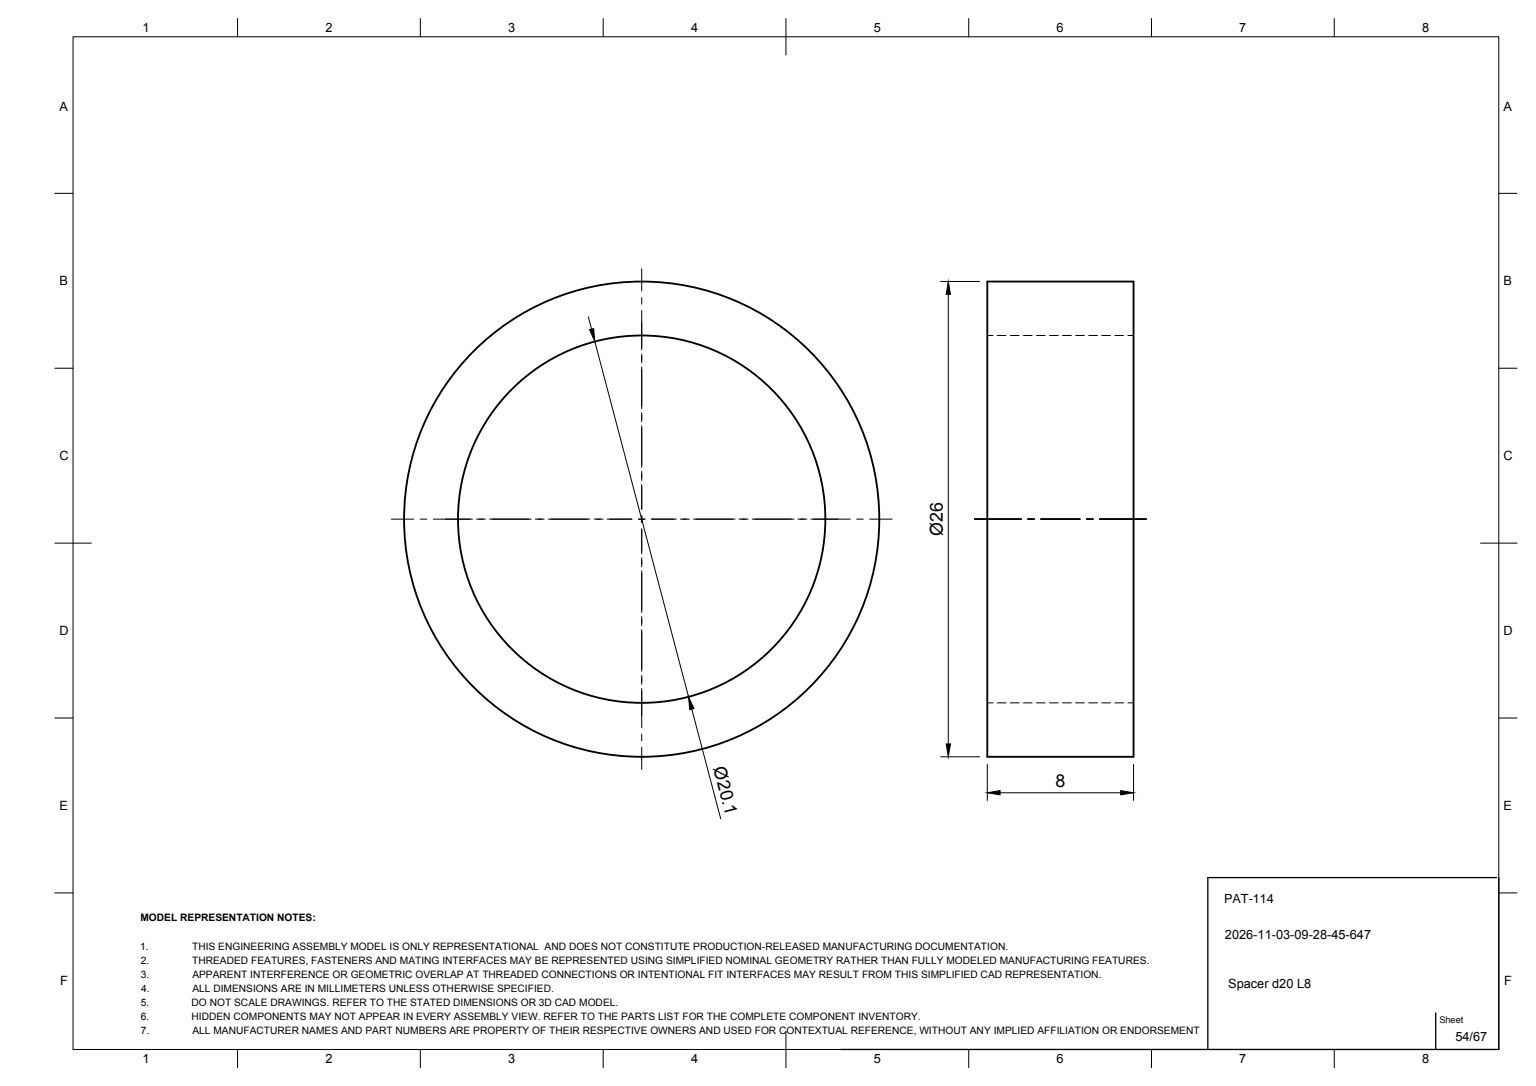
ISO-10303-21;
HEADER;
/* Generated by software containing ST-Developer
 * from STEP Tools, Inc. (www.steptools.com) 
 */

FILE_DESCRIPTION(
/* description */ ('Two-stage gear reducer in split housing'),
/* implementation_level */ '2;1');

FILE_NAME(
/* name */ 'Spacer d20 L8.step',
/* time_stamp */ '2026-10-28T03:22:31-07:00',
/* author */ (''),
/* organization */ (''),
/* preprocessor_version */ 'ST-DEVELOPER v20.2',
/* originating_system */ 'Autodesk Translation Framework v15.17.0.0',
/* authorisation */ '');

FILE_SCHEMA (('AUTOMOTIVE_DESIGN { 1 0 10303 214 3 1 1 }'));
ENDSEC;

DATA;
#10=MECHANICAL_DESIGN_GEOMETRIC_PRESENTATION_REPRESENTATION('',(#1292),#73366);
#1165=SHAPE_REPRESENTATION_RELATIONSHIP('SRR','None',#73656,#1221);
#1221=ADVANCED_BREP_SHAPE_REPRESENTATION('',(#1361),#73352);
#1292=STYLED_ITEM('',(#73981),#1361);
#1361=MANIFOLD_SOLID_BREP('Body1',#16182);
#1574=FACE_BOUND('',#3707,.T.);
#1575=FACE_BOUND('',#3709,.T.);
#1884=PLANE('',#18033);
#1885=PLANE('',#18034);
#2591=FACE_OUTER_BOUND('',#3704,.T.);
#2592=FACE_OUTER_BOUND('',#3705,.T.);
#2593=FACE_OUTER_BOUND('',#3706,.T.);
#2594=FACE_OUTER_BOUND('',#3708,.T.);
#3704=EDGE_LOOP('',(#13143,#13144,#13145,#13146));
#3705=EDGE_LOOP('',(#13147,#13148,#13149,#13150));
#3706=EDGE_LOOP('',(#13151));
#3707=EDGE_LOOP('',(#13152));
#3708=EDGE_LOOP('',(#13153));
#3709=EDGE_LOOP('',(#13154));
#4700=LINE('',#37636,#5724);
#4701=LINE('',#37642,#5725);
#5724=VECTOR('',#21536,1.005);
#5725=VECTOR('',#21543,1.3);
#6650=CIRCLE('',#18028,1.005);
#6651=CIRCLE('',#18029,1.005);
#6652=CIRCLE('',#18031,1.3);
#6653=CIRCLE('',#18032,1.3);
#7719=VERTEX_POINT('',#37633);
#7720=VERTEX_POINT('',#37635);
#7721=VERTEX_POINT('',#37639);
#7722=VERTEX_POINT('',#37641);
#9625=EDGE_CURVE('',#7719,#7719,#6650,.T.);
#9626=EDGE_CURVE('',#7719,#7720,#4700,.T.);
#9627=EDGE_CURVE('',#7720,#7720,#6651,.T.);
#9628=EDGE_CURVE('',#7721,#7721,#6652,.T.);
#9629=EDGE_CURVE('',#7721,#7722,#4701,.T.);
#9630=EDGE_CURVE('',#7722,#7722,#6653,.T.);
#13143=ORIENTED_EDGE('',*,*,#9625,.F.);
#13144=ORIENTED_EDGE('',*,*,#9626,.T.);
#13145=ORIENTED_EDGE('',*,*,#9627,.T.);
#13146=ORIENTED_EDGE('',*,*,#9626,.F.);
#13147=ORIENTED_EDGE('',*,*,#9628,.F.);
#13148=ORIENTED_EDGE('',*,*,#9629,.T.);
#13149=ORIENTED_EDGE('',*,*,#9630,.T.);
#13150=ORIENTED_EDGE('',*,*,#9629,.F.);
#13151=ORIENTED_EDGE('',*,*,#9628,.T.);
#13152=ORIENTED_EDGE('',*,*,#9625,.T.);
#13153=ORIENTED_EDGE('',*,*,#9630,.F.);
#13154=ORIENTED_EDGE('',*,*,#9627,.F.);
#15125=CYLINDRICAL_SURFACE('',#18027,1.005);
#15126=CYLINDRICAL_SURFACE('',#18030,1.3);
#15798=ADVANCED_FACE('',(#2591),#15125,.F.);
#15799=ADVANCED_FACE('',(#2592),#15126,.T.);
#15800=ADVANCED_FACE('',(#2593,#1574),#1884,.T.);
#15801=ADVANCED_FACE('',(#2594,#1575),#1885,.F.);
#16182=CLOSED_SHELL('',(#15798,#15799,#15800,#15801));
#18026=AXIS2_PLACEMENT_3D('',#37631,#21530,#21531);
#18027=AXIS2_PLACEMENT_3D('',#37632,#21532,#21533);
#18028=AXIS2_PLACEMENT_3D('',#37634,#21534,#21535);
#18029=AXIS2_PLACEMENT_3D('',#37637,#21537,#21538);
#18030=AXIS2_PLACEMENT_3D('',#37638,#21539,#21540);
#18031=AXIS2_PLACEMENT_3D('',#37640,#21541,#21542);
#18032=AXIS2_PLACEMENT_3D('',#37643,#21544,#21545);
#18033=AXIS2_PLACEMENT_3D('',#37644,#21546,#21547);
#18034=AXIS2_PLACEMENT_3D('',#37645,#21548,#21549);
#21530=DIRECTION('axis',(0.,0.,1.));
#21531=DIRECTION('refdir',(1.,0.,0.));
#21532=DIRECTION('center_axis',(0.,1.,0.));
#21533=DIRECTION('ref_axis',(1.,0.,0.));
#21534=DIRECTION('center_axis',(0.,-1.,0.));
#21535=DIRECTION('ref_axis',(1.,0.,0.));
#21536=DIRECTION('',(0.,-1.,0.));
#21537=DIRECTION('center_axis',(0.,-1.,0.));
#21538=DIRECTION('ref_axis',(1.,0.,0.));
#21539=DIRECTION('center_axis',(0.,1.,0.));
#21540=DIRECTION('ref_axis',(1.,0.,0.));
#21541=DIRECTION('center_axis',(0.,1.,0.));
#21542=DIRECTION('ref_axis',(1.,0.,0.));
#21543=DIRECTION('',(0.,-1.,0.));
#21544=DIRECTION('center_axis',(0.,1.,0.));
#21545=DIRECTION('ref_axis',(1.,0.,0.));
#21546=DIRECTION('center_axis',(0.,1.,0.));
#21547=DIRECTION('ref_axis',(1.,0.,0.));
#21548=DIRECTION('center_axis',(0.,1.,0.));
#21549=DIRECTION('ref_axis',(1.,0.,0.));
#37631=CARTESIAN_POINT('',(0.,0.,0.));
#37632=CARTESIAN_POINT('Origin',(6.,0.2,10.));
#37633=CARTESIAN_POINT('',(4.995,1.,10.));
#37634=CARTESIAN_POINT('Origin',(6.,1.,10.));
#37635=CARTESIAN_POINT('',(4.995,0.2,10.));
#37636=CARTESIAN_POINT('',(4.995,0.2,10.));
#37637=CARTESIAN_POINT('Origin',(6.,0.2,10.));
#37638=CARTESIAN_POINT('Origin',(6.,0.2,10.));
#37639=CARTESIAN_POINT('',(4.7,1.,10.));
#37640=CARTESIAN_POINT('Origin',(6.,1.,10.));
#37641=CARTESIAN_POINT('',(4.7,0.2,10.));
#37642=CARTESIAN_POINT('',(4.7,0.2,10.));
#37643=CARTESIAN_POINT('Origin',(6.,0.2,10.));
#37644=CARTESIAN_POINT('Origin',(6.,1.,10.));
#37645=CARTESIAN_POINT('Origin',(6.,0.2,10.));
#73288=UNCERTAINTY_MEASURE_WITH_UNIT(LENGTH_MEASURE(0.001),#73367,
'DISTANCE_ACCURACY_VALUE',
'Maximum model space distance between geometric entities at asserted c
onnectivities');
#73302=UNCERTAINTY_MEASURE_WITH_UNIT(LENGTH_MEASURE(0.001),#73367,
'DISTANCE_ACCURACY_VALUE',
'Maximum model space distance between geometric entities at asserted c
onnectivities');
#73352=(
GEOMETRIC_REPRESENTATION_CONTEXT(3)
GLOBAL_UNCERTAINTY_ASSIGNED_CONTEXT((#73288))
GLOBAL_UNIT_ASSIGNED_CONTEXT((#73367,#73369,#73370))
REPRESENTATION_CONTEXT('','3D')
);
#73366=(
GEOMETRIC_REPRESENTATION_CONTEXT(3)
GLOBAL_UNCERTAINTY_ASSIGNED_CONTEXT((#73302))
GLOBAL_UNIT_ASSIGNED_CONTEXT((#73367,#73369,#73370))
REPRESENTATION_CONTEXT('','3D')
);
#73367=(
LENGTH_UNIT()
NAMED_UNIT(*)
SI_UNIT(.CENTI.,.METRE.)
);
#73369=(
NAMED_UNIT(*)
PLANE_ANGLE_UNIT()
SI_UNIT($,.RADIAN.)
);
#73370=(
NAMED_UNIT(*)
SI_UNIT($,.STERADIAN.)
SOLID_ANGLE_UNIT()
);
#73420=SHAPE_DEFINITION_REPRESENTATION(#73553,#73656);
#73553=PRODUCT_DEFINITION_SHAPE('',$,#73720);
#73656=SHAPE_REPRESENTATION('',(#18026),#73352);
#73670=PRODUCT_DEFINITION_CONTEXT('part definition',#73861,'design');
#73720=PRODUCT_DEFINITION('Spacer d20 L8','Spacer d20 L8',#73783,#73670);
#73783=PRODUCT_DEFINITION_FORMATION('',$,#73912);
#73861=APPLICATION_CONTEXT(
'Core Data for Automotive Mechanical Design Process');
#73862=PRODUCT_CONTEXT('part definition',#73861,'mechanical');
#73912=PRODUCT('Spacer d20 L8','Spacer d20 L8','Spacer d20 L8',(#73862));
#73975=COLOUR_RGB('Sky Blue',0.24,0.69,0.87);
#73976=FILL_AREA_STYLE_COLOUR('',#73975);
#73977=FILL_AREA_STYLE('',(#73976));
#73978=SURFACE_STYLE_FILL_AREA(#73977);
#73979=SURFACE_SIDE_STYLE('',(#73978));
#73980=SURFACE_STYLE_USAGE(.BOTH.,#73979);
#73981=PRESENTATION_STYLE_ASSIGNMENT((#73980));
ENDSEC;
END-ISO-10303-21;
